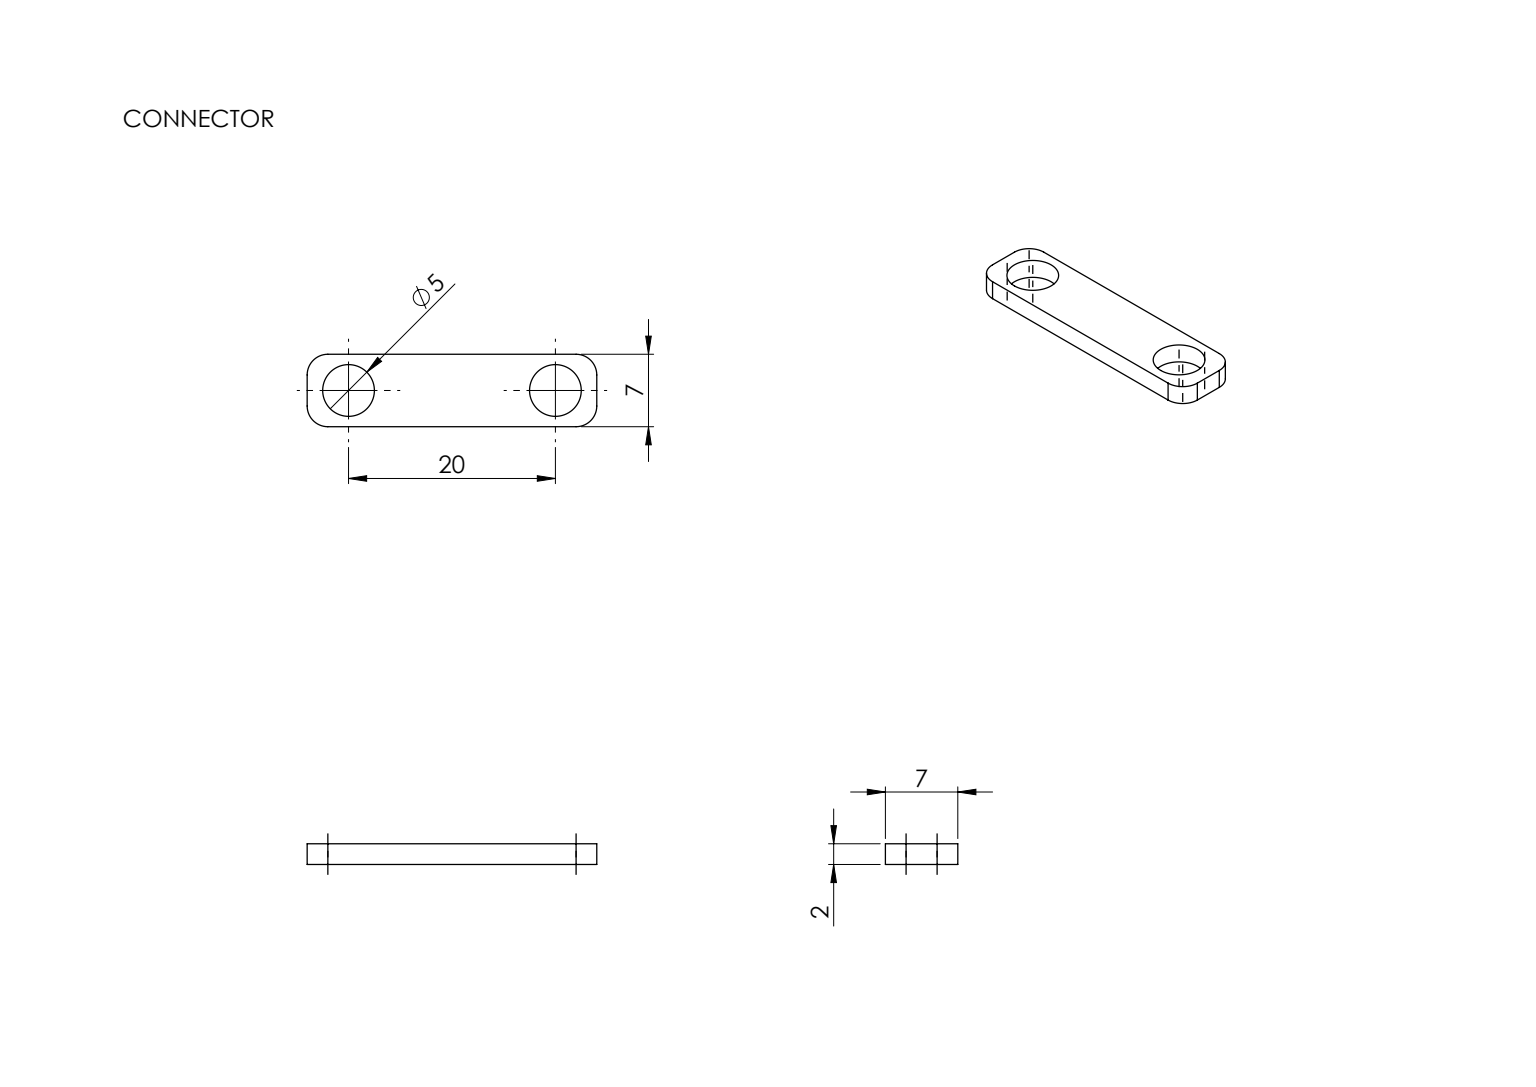
ISO-10303-21;
HEADER;
FILE_DESCRIPTION (('STEP AP214'),
    '1' );
FILE_NAME ('connector.step',
    '2026-10-08T13:56:24',
    ( '' ),
    ( '' ),
    'SwSTEP 2.0',
    'SolidWorks 2026',
    '' );
FILE_SCHEMA (( 'AUTOMOTIVE_DESIGN' ));
ENDSEC;

DATA;
#18=ADVANCED_FACE ( 'NONE', ( #40 ), #4954, .F. ) ;
#25=DIRECTION ( 'NONE',  ( -0.000000000000000000, -1.000000000000000000, -0.000000000000000000 ) ) ;
#35=LINE ( 'NONE', #1227, #14934 ) ;
#40=FACE_OUTER_BOUND ( 'NONE', #10361, .T. ) ;
#55=ORIENTED_EDGE ( 'NONE', *, *, #1011, .T. ) ;
#119=EDGE_CURVE ( 'NONE', #13173, #1506, #10244, .T. ) ;
#142=AXIS2_PLACEMENT_3D ( 'NONE', #6437, #6586, #9027 ) ;
#156=DIRECTION ( 'NONE',  ( 0.000000000000000000, 1.000000000000000000, -0.000000000000000000 ) ) ;
#158=ORIENTED_EDGE ( 'NONE', *, *, #11026, .F. ) ;
#174=PLANE ( 'NONE',  #5147 ) ;
#229=ORIENTED_EDGE ( 'NONE', *, *, #1759, .F. ) ;
#241=VECTOR ( 'NONE', #6289, 1000.000000000000000 ) ;
#307=VERTEX_POINT ( 'NONE', #7662 ) ;
#454=ORIENTED_EDGE ( 'NONE', *, *, #5990, .F. ) ;
#498=DIRECTION ( 'NONE',  ( 1.000000000000000000, 0.000000000000000000, 0.000000000000000000 ) ) ;
#522=VECTOR ( 'NONE', #25, 1000.000000000000000 ) ;
#523=FACE_OUTER_BOUND ( 'NONE', #7763, .T. ) ;
#595=FILL_AREA_STYLE_COLOUR ( '', #11712 ) ;
#608=ADVANCED_BREP_SHAPE_REPRESENTATION ( '', ( #9113, #3223 ), #1938 ) ;
#618=CARTESIAN_POINT ( 'NONE',  ( -17.99999999999979394, -11.00000000000000178, 1.499999999999999112 ) ) ;
#684=CIRCLE ( 'NONE', #4805, 2.000000000000000888 ) ;
#698=DIRECTION ( 'NONE',  ( 0.000000000000000000, 0.000000000000000000, 1.000000000000000000 ) ) ;
#724=AXIS2_PLACEMENT_3D ( 'NONE', #13932, #9982, #2858 ) ;
#756=PRESENTATION_STYLE_ASSIGNMENT (( #11957 ) ) ;
#763=ADVANCED_FACE ( 'NONE', ( #6395 ), #15112, .T. ) ;
#800=EDGE_CURVE ( 'NONE', #4542, #3229, #6635, .T. ) ;
#828=( NAMED_UNIT ( * ) PLANE_ANGLE_UNIT ( ) SI_UNIT ( $, .RADIAN. ) );
#835=CARTESIAN_POINT ( 'NONE',  ( -39.99999999999999289, -11.00000000000000178, 2.500000000001739497 ) ) ;
#849=ORIENTED_EDGE ( 'NONE', *, *, #13885, .T. ) ;
#862=FILL_AREA_STYLE_COLOUR ( '', #3052 ) ;
#897=ORIENTED_EDGE ( 'NONE', *, *, #7225, .T. ) ;
#914=CYLINDRICAL_SURFACE ( 'NONE', #5036, 2.500000000000909495 ) ;
#968=EDGE_LOOP ( 'NONE', ( #5323, #8194, #3762, #2718 ) ) ;
#1005=CYLINDRICAL_SURFACE ( 'NONE', #2041, 2.499999999999998668 ) ;
#1010=CARTESIAN_POINT ( 'NONE',  ( -19.99999999999956657, -11.00000000000000178, 8.786575603324269439E-13 ) ) ;
#1011=EDGE_CURVE ( 'NONE', #9125, #9091, #1099, .T. ) ;
#1051=LINE ( 'NONE', #12031, #10121 ) ;
#1087=SURFACE_SIDE_STYLE ('',( #12150 ) ) ;
#1099=CIRCLE ( 'NONE', #8348, 2.000000000000000888 ) ;
#1133=ORIENTED_EDGE ( 'NONE', *, *, #3684, .T. ) ;
#1158=CARTESIAN_POINT ( 'NONE',  ( -19.99999999999956657, -11.00000000000000178, -2.499999999999120259 ) ) ;
#1164=CARTESIAN_POINT ( 'NONE',  ( -15.99999999999979217, -9.000000000000001776, -1.500000000000001110 ) ) ;
#1180=EDGE_CURVE ( 'NONE', #9048, #13189, #4457, .T. ) ;
#1193=ORIENTED_EDGE ( 'NONE', *, *, #1975, .T. ) ;
#1227=CARTESIAN_POINT ( 'NONE',  ( -41.99999999999978684, -11.00000000000000178, 3.499999999999998668 ) ) ;
#1254=ORIENTED_EDGE ( 'NONE', *, *, #1180, .T. ) ;
#1305=DIRECTION ( 'NONE',  ( 0.000000000000000000, 0.000000000000000000, 1.000000000000000000 ) ) ;
#1385=CARTESIAN_POINT ( 'NONE',  ( -39.99999999999999289, -9.000000000000001776, 8.300651832549021947E-13 ) ) ;
#1476=VERTEX_POINT ( 'NONE', #4588 ) ;
#1506=VERTEX_POINT ( 'NONE', #15355 ) ;
#1518=VECTOR ( 'NONE', #3284, 1000.000000000000000 ) ;
#1677=CARTESIAN_POINT ( 'NONE',  ( -41.99999999999978684, -11.00000000000000178, 1.499999999999999112 ) ) ;
#1692=FACE_OUTER_BOUND ( 'NONE', #5404, .T. ) ;
#1707=DIRECTION ( 'NONE',  ( 0.000000000000000000, 0.000000000000000000, 1.000000000000000000 ) ) ;
#1759=EDGE_CURVE ( 'NONE', #1476, #14724, #14936, .T. ) ;
#1818=DIRECTION ( 'NONE',  ( 0.000000000000000000, 0.000000000000000000, -1.000000000000000000 ) ) ;
#1868=( NAMED_UNIT ( * ) SI_UNIT ( $, .STERADIAN. ) SOLID_ANGLE_UNIT ( ) );
#1880=CARTESIAN_POINT ( 'NONE',  ( -39.99999999999999289, -9.000000000000001776, -2.500000000000079492 ) ) ;
#1938=( GEOMETRIC_REPRESENTATION_CONTEXT ( 3 ) GLOBAL_UNCERTAINTY_ASSIGNED_CONTEXT ( ( #7400 ) ) GLOBAL_UNIT_ASSIGNED_CONTEXT ( ( #14406, #828, #1868 ) ) REPRESENTATION_CONTEXT ( 'NONE', 'WORKASPACE' ) );
#1957=APPLICATION_CONTEXT ( 'automotive_design' ) ;
#1961=VECTOR ( 'NONE', #15902, 1000.000000000000000 ) ;
#1974=ORIENTED_EDGE ( 'NONE', *, *, #5141, .T. ) ;
#1975=EDGE_CURVE ( 'NONE', #6779, #6035, #6277, .T. ) ;
#1985=CARTESIAN_POINT ( 'NONE',  ( -41.99999999999978684, -9.000000000000001776, 3.499999999999998668 ) ) ;
#2039=DIRECTION ( 'NONE',  ( 0.000000000000000000, 0.000000000000000000, 1.000000000000000000 ) ) ;
#2041=AXIS2_PLACEMENT_3D ( 'NONE', #9494, #3190, #14264 ) ;
#2057=ORIENTED_EDGE ( 'NONE', *, *, #7517, .T. ) ;
#2073=ORIENTED_EDGE ( 'NONE', *, *, #7225, .F. ) ;
#2109=ORIENTED_EDGE ( 'NONE', *, *, #5990, .T. ) ;
#2140=CARTESIAN_POINT ( 'NONE',  ( -17.99999999999979394, -9.000000000000001776, -3.500000000000000888 ) ) ;
#2146=EDGE_LOOP ( 'NONE', ( #849, #3533 ) ) ;
#2166=EDGE_LOOP ( 'NONE', ( #10473, #8805 ) ) ;
#2254=DIRECTION ( 'NONE',  ( 0.000000000000000000, 0.000000000000000000, 1.000000000000000000 ) ) ;
#2269=MECHANICAL_DESIGN_GEOMETRIC_PRESENTATION_REPRESENTATION('',(#9256),#10548);
#2317=LINE ( 'NONE', #3611, #13079 ) ;
#2336=CARTESIAN_POINT ( 'NONE',  ( -39.99999999999999289, -11.00000000000000178, 8.300651832549021947E-13 ) ) ;
#2350=EDGE_CURVE ( 'NONE', #307, #2847, #1051, .T. ) ;
#2464=CARTESIAN_POINT ( 'NONE',  ( -15.99999999999979217, -9.000000000000001776, -1.500000000000001110 ) ) ;
#2554=CARTESIAN_POINT ( 'NONE',  ( -41.99999999999978684, -11.00000000000000178, -3.500000000000001776 ) ) ;
#2659=EDGE_CURVE ( 'NONE', #2847, #3269, #15607, .T. ) ;
#2701=FACE_BOUND ( 'NONE', #2146, .T. ) ;
#2718=ORIENTED_EDGE ( 'NONE', *, *, #5141, .F. ) ;
#2728=CARTESIAN_POINT ( 'NONE',  ( -17.99999999999979394, -9.000000000000001776, 1.499999999999999112 ) ) ;
#2847=VERTEX_POINT ( 'NONE', #2554 ) ;
#2858=DIRECTION ( 'NONE',  ( 0.000000000000000000, 0.000000000000000000, 1.000000000000000000 ) ) ;
#2860=DIRECTION ( 'NONE',  ( 0.000000000000000000, -0.000000000000000000, 1.000000000000000000 ) ) ;
#2875=CARTESIAN_POINT ( 'NONE',  ( -15.99999999999979217, -11.00000000000000178, -1.500000000000001110 ) ) ;
#2886=ORIENTED_EDGE ( 'NONE', *, *, #14291, .F. ) ;
#2928=LINE ( 'NONE', #1880, #7434 ) ;
#2937=DIRECTION ( 'NONE',  ( 0.000000000000000000, 1.000000000000000000, 0.000000000000000000 ) ) ;
#2945=FACE_OUTER_BOUND ( 'NONE', #968, .T. ) ;
#3005=ORIENTED_EDGE ( 'NONE', *, *, #1011, .F. ) ;
#3013=CARTESIAN_POINT ( 'NONE',  ( -15.99999999999979217, -9.000000000000001776, -1.500000000000001110 ) ) ;
#3034=FACE_OUTER_BOUND ( 'NONE', #10178, .T. ) ;
#3052=COLOUR_RGB ( '', 0.40784314, 0.44705882, 0.49803922) ;
#3102=EDGE_CURVE ( 'NONE', #12397, #3134, #14026, .T. ) ;
#3110=DIRECTION ( 'NONE',  ( 1.000000000000000000, 0.000000000000000000, 0.000000000000000000 ) ) ;
#3134=VERTEX_POINT ( 'NONE', #10577 ) ;
#3190=DIRECTION ( 'NONE',  ( -0.000000000000000000, -1.000000000000000000, -0.000000000000000000 ) ) ;
#3223=AXIS2_PLACEMENT_3D ( 'NONE', #11897, #11972, #4638 ) ;
#3229=VERTEX_POINT ( 'NONE', #10485 ) ;
#3239=DIRECTION ( 'NONE',  ( 0.000000000000000000, 1.000000000000000000, -0.000000000000000000 ) ) ;
#3256=CYLINDRICAL_SURFACE ( 'NONE', #6862, 2.000000000000000888 ) ;
#3269=VERTEX_POINT ( 'NONE', #12966 ) ;
#3276=CARTESIAN_POINT ( 'NONE',  ( -39.99999999999999289, -9.000000000000001776, 8.300651832549021947E-13 ) ) ;
#3284=DIRECTION ( 'NONE',  ( -0.000000000000000000, -1.000000000000000000, -0.000000000000000000 ) ) ;
#3332=ADVANCED_FACE ( 'NONE', ( #7249 ), #12072, .F. ) ;
#3402=FILL_AREA_STYLE ('',( #595 ) ) ;
#3413=DIRECTION ( 'NONE',  ( -0.000000000000000000, -1.000000000000000000, -0.000000000000000000 ) ) ;
#3428=DIRECTION ( 'NONE',  ( 0.000000000000000000, 1.000000000000000000, 0.000000000000000000 ) ) ;
#3469=DIRECTION ( 'NONE',  ( -1.000000000000000000, -0.000000000000000000, -0.000000000000000000 ) ) ;
#3499=DIRECTION ( 'NONE',  ( 0.000000000000000000, 0.000000000000000000, 1.000000000000000000 ) ) ;
#3518=AXIS2_PLACEMENT_3D ( 'NONE', #7554, #14986, #4060 ) ;
#3533=ORIENTED_EDGE ( 'NONE', *, *, #5671, .T. ) ;
#3607=LINE ( 'NONE', #7100, #1961 ) ;
#3611=CARTESIAN_POINT ( 'NONE',  ( -15.99999999999979217, -9.000000000000001776, -1.500000000000001110 ) ) ;
#3684=EDGE_CURVE ( 'NONE', #10705, #12397, #9407, .T. ) ;
#3762=ORIENTED_EDGE ( 'NONE', *, *, #14528, .F. ) ;
#3786=VECTOR ( 'NONE', #7903, 1000.000000000000000 ) ;
#3809=CIRCLE ( 'NONE', #724, 2.000000000000000888 ) ;
#3810=ADVANCED_FACE ( 'NONE', ( #7468, #13914, #7548 ), #3892, .T. ) ;
#3833=PRODUCT_DEFINITION_CONTEXT ( 'detailed design', #1957, 'design' ) ;
#3846=ORIENTED_EDGE ( 'NONE', *, *, #7499, .T. ) ;
#3872=CYLINDRICAL_SURFACE ( 'NONE', #14600, 2.000000000000000888 ) ;
#3892=PLANE ( 'NONE',  #8955 ) ;
#3893=DIRECTION ( 'NONE',  ( -0.000000000000000000, -1.000000000000000000, -0.000000000000000000 ) ) ;
#3897=CARTESIAN_POINT ( 'NONE',  ( -41.99999999999978684, -9.000000000000001776, 3.499999999999998668 ) ) ;
#3902=EDGE_CURVE ( 'NONE', #6035, #6779, #12054, .T. ) ;
#3941=DIRECTION ( 'NONE',  ( 0.000000000000000000, 0.000000000000000000, 1.000000000000000000 ) ) ;
#4031=ADVANCED_FACE ( 'NONE', ( #523 ), #5678, .T. ) ;
#4046=LINE ( 'NONE', #8917, #4614 ) ;
#4060=DIRECTION ( 'NONE',  ( 0.000000000000000000, 0.000000000000000000, 1.000000000000000000 ) ) ;
#4065=FACE_OUTER_BOUND ( 'NONE', #7295, .T. ) ;
#4156=FACE_BOUND ( 'NONE', #2166, .T. ) ;
#4179=UNCERTAINTY_MEASURE_WITH_UNIT (LENGTH_MEASURE( 1.000000000000000082E-05 ), #14586, 'distance_accuracy_value', 'NONE');
#4242=ORIENTED_EDGE ( 'NONE', *, *, #13940, .F. ) ;
#4263=AXIS2_PLACEMENT_3D ( 'NONE', #618, #2937, #2860 ) ;
#4292=ORIENTED_EDGE ( 'NONE', *, *, #3102, .T. ) ;
#4381=EDGE_CURVE ( 'NONE', #9125, #14724, #2317, .T. ) ;
#4410=ORIENTED_EDGE ( 'NONE', *, *, #9663, .F. ) ;
#4419=CARTESIAN_POINT ( 'NONE',  ( -19.99999999999956657, -9.000000000000001776, -2.499999999999120259 ) ) ;
#4426=ORIENTED_EDGE ( 'NONE', *, *, #800, .T. ) ;
#4457=CIRCLE ( 'NONE', #11675, 2.499999999999998668 ) ;
#4466=ORIENTED_EDGE ( 'NONE', *, *, #7538, .F. ) ;
#4528=AXIS2_PLACEMENT_3D ( 'NONE', #15021, #156, #9842 ) ;
#4542=VERTEX_POINT ( 'NONE', #12721 ) ;
#4588=CARTESIAN_POINT ( 'NONE',  ( -15.99999999999979217, -11.00000000000000178, 1.499999999999998890 ) ) ;
#4602=EDGE_CURVE ( 'NONE', #9091, #13173, #9194, .T. ) ;
#4614=VECTOR ( 'NONE', #1707, 1000.000000000000000 ) ;
#4619=AXIS2_PLACEMENT_3D ( 'NONE', #5093, #12506, #6633 ) ;
#4622=SURFACE_SIDE_STYLE ('',( #5519 ) ) ;
#4638=DIRECTION ( 'NONE',  ( 1.000000000000000000, 0.000000000000000000, 0.000000000000000000 ) ) ;
#4656=ORIENTED_EDGE ( 'NONE', *, *, #7809, .T. ) ;
#4735=ORIENTED_EDGE ( 'NONE', *, *, #9375, .F. ) ;
#4783=CIRCLE ( 'NONE', #5813, 2.499999999999998668 ) ;
#4784=CARTESIAN_POINT ( 'NONE',  ( -39.99999999999999289, -9.000000000000001776, 8.300651832549021947E-13 ) ) ;
#4805=AXIS2_PLACEMENT_3D ( 'NONE', #1677, #8808, #3941 ) ;
#4866=CIRCLE ( 'NONE', #15198, 2.500000000000909495 ) ;
#4878=DIRECTION ( 'NONE',  ( 1.000000000000000000, 0.000000000000000000, 0.000000000000000000 ) ) ;
#4954=CYLINDRICAL_SURFACE ( 'NONE', #8447, 2.499999999999998668 ) ;
#4984=CARTESIAN_POINT ( 'NONE',  ( -17.99999999999979394, -9.000000000000001776, -3.500000000000000888 ) ) ;
#5036=AXIS2_PLACEMENT_3D ( 'NONE', #4784, #5756, #7297 ) ;
#5093=CARTESIAN_POINT ( 'NONE',  ( -17.99999999999979394, -11.00000000000000178, 1.499999999999999112 ) ) ;
#5141=EDGE_CURVE ( 'NONE', #6035, #9656, #2928, .T. ) ;
#5147=AXIS2_PLACEMENT_3D ( 'NONE', #5421, #498, #10274 ) ;
#5156=LINE ( 'NONE', #11441, #241 ) ;
#5227=AXIS2_PLACEMENT_3D ( 'NONE', #6476, #7697, #10426 ) ;
#5253=DIRECTION ( 'NONE',  ( -0.000000000000000000, -1.000000000000000000, -0.000000000000000000 ) ) ;
#5297=ORIENTED_EDGE ( 'NONE', *, *, #1180, .F. ) ;
#5323=ORIENTED_EDGE ( 'NONE', *, *, #3902, .T. ) ;
#5404=EDGE_LOOP ( 'NONE', ( #897, #6728, #8945, #4656 ) ) ;
#5421=CARTESIAN_POINT ( 'NONE',  ( -43.99999999999978684, -9.000000000000001776, -1.500000000000000666 ) ) ;
#5429=ORIENTED_EDGE ( 'NONE', *, *, #7499, .F. ) ;
#5431=VERTEX_POINT ( 'NONE', #8148 ) ;
#5433=EDGE_CURVE ( 'NONE', #10705, #11234, #13045, .T. ) ;
#5440=DIRECTION ( 'NONE',  ( -0.000000000000000000, -1.000000000000000000, -0.000000000000000000 ) ) ;
#5481=ORIENTED_EDGE ( 'NONE', *, *, #9501, .T. ) ;
#5516=CARTESIAN_POINT ( 'NONE',  ( -41.99999999999978684, -9.000000000000001776, -1.500000000000000888 ) ) ;
#5519=SURFACE_STYLE_FILL_AREA ( #3402 ) ;
#5542=ORIENTED_EDGE ( 'NONE', *, *, #13940, .T. ) ;
#5617=CARTESIAN_POINT ( 'NONE',  ( -39.99999999999999289, -9.000000000000001776, -2.500000000000079492 ) ) ;
#5624=DIRECTION ( 'NONE',  ( 1.000000000000000000, 0.000000000000000000, -0.000000000000000000 ) ) ;
#5671=EDGE_CURVE ( 'NONE', #11827, #6744, #9496, .T. ) ;
#5678=CYLINDRICAL_SURFACE ( 'NONE', #14145, 2.000000000000000888 ) ;
#5756=DIRECTION ( 'NONE',  ( -0.000000000000000000, -1.000000000000000000, -0.000000000000000000 ) ) ;
#5813=AXIS2_PLACEMENT_3D ( 'NONE', #8537, #14577, #3499 ) ;
#5832=SHAPE_REPRESENTATION_RELATIONSHIP ( 'NONE' , 'NONE' ,  #15130, #608 ) ;
#5843=AXIS2_PLACEMENT_3D ( 'NONE', #3276, #6764, #1818 ) ;
#5906=VECTOR ( 'NONE', #3893, 1000.000000000000000 ) ;
#5910=AXIS2_PLACEMENT_3D ( 'NONE', #14748, #13275, #8618 ) ;
#5990=EDGE_CURVE ( 'NONE', #4542, #10705, #3809, .T. ) ;
#6027=( NAMED_UNIT ( * ) SI_UNIT ( $, .STERADIAN. ) SOLID_ANGLE_UNIT ( ) );
#6035=VERTEX_POINT ( 'NONE', #5617 ) ;
#6036=PRODUCT ( 'connector', 'connector', '', ( #7465 ) ) ;
#6108=PRESENTATION_STYLE_ASSIGNMENT (( #10870 ) ) ;
#6186=DIRECTION ( 'NONE',  ( 0.000000000000000000, 0.000000000000000000, 1.000000000000000000 ) ) ;
#6237=EDGE_CURVE ( 'NONE', #11234, #3134, #35, .T. ) ;
#6251=DIRECTION ( 'NONE',  ( 0.000000000000000000, -0.000000000000000000, 1.000000000000000000 ) ) ;
#6276=EDGE_LOOP ( 'NONE', ( #15549, #12998, #5429, #5481 ) ) ;
#6277=CIRCLE ( 'NONE', #15310, 2.500000000000909495 ) ;
#6289=DIRECTION ( 'NONE',  ( -0.000000000000000000, -1.000000000000000000, -0.000000000000000000 ) ) ;
#6395=FACE_OUTER_BOUND ( 'NONE', #14036, .T. ) ;
#6408=AXIS2_PLACEMENT_3D ( 'NONE', #1385, #13740, #1305 ) ;
#6437=CARTESIAN_POINT ( 'NONE',  ( -39.99999999999999289, -11.00000000000000178, 8.300651832549021947E-13 ) ) ;
#6476=CARTESIAN_POINT ( 'NONE',  ( -41.99999999999978684, -9.000000000000001776, 1.499999999999999112 ) ) ;
#6516=EDGE_LOOP ( 'NONE', ( #5297, #4242 ) ) ;
#6529=VECTOR ( 'NONE', #14023, 1000.000000000000000 ) ;
#6586=DIRECTION ( 'NONE',  ( 0.000000000000000000, 1.000000000000000000, 0.000000000000000000 ) ) ;
#6607=DIRECTION ( 'NONE',  ( -0.000000000000000000, -1.000000000000000000, -0.000000000000000000 ) ) ;
#6624=DIRECTION ( 'NONE',  ( -0.000000000000000000, -1.000000000000000000, -0.000000000000000000 ) ) ;
#6633=DIRECTION ( 'NONE',  ( 0.000000000000000000, 0.000000000000000000, 1.000000000000000000 ) ) ;
#6635=LINE ( 'NONE', #13896, #12964 ) ;
#6668=PLANE ( 'NONE',  #12255 ) ;
#6723=PRODUCT_DEFINITION ( 'UNKNOWN', '', #8973, #3833 ) ;
#6728=ORIENTED_EDGE ( 'NONE', *, *, #800, .F. ) ;
#6744=VERTEX_POINT ( 'NONE', #1158 ) ;
#6764=DIRECTION ( 'NONE',  ( -0.000000000000000000, -1.000000000000000000, -0.000000000000000000 ) ) ;
#6779=VERTEX_POINT ( 'NONE', #11029 ) ;
#6811=ORIENTED_EDGE ( 'NONE', *, *, #4602, .F. ) ;
#6812=( NAMED_UNIT ( * ) PLANE_ANGLE_UNIT ( ) SI_UNIT ( $, .RADIAN. ) );
#6831=ORIENTED_EDGE ( 'NONE', *, *, #9501, .F. ) ;
#6833=ORIENTED_EDGE ( 'NONE', *, *, #2350, .T. ) ;
#6862=AXIS2_PLACEMENT_3D ( 'NONE', #11494, #15552, #10620 ) ;
#6904=DIRECTION ( 'NONE',  ( 0.000000000000000000, 0.000000000000000000, 1.000000000000000000 ) ) ;
#6931=DIRECTION ( 'NONE',  ( -0.000000000000000000, -1.000000000000000000, -0.000000000000000000 ) ) ;
#6945=ORIENTED_EDGE ( 'NONE', *, *, #5671, .F. ) ;
#6965=VERTEX_POINT ( 'NONE', #835 ) ;
#6995=ORIENTED_EDGE ( 'NONE', *, *, #11649, .T. ) ;
#6998=EDGE_LOOP ( 'NONE', ( #1254, #7541, #7678, #4735 ) ) ;
#7009=CARTESIAN_POINT ( 'NONE',  ( -43.99999999999978684, -9.000000000000001776, -1.500000000000000666 ) ) ;
#7095=ORIENTED_EDGE ( 'NONE', *, *, #5433, .T. ) ;
#7100=CARTESIAN_POINT ( 'NONE',  ( -39.99999999999999289, -9.000000000000001776, 2.500000000001739497 ) ) ;
#7199=ORIENTED_EDGE ( 'NONE', *, *, #119, .F. ) ;
#7225=EDGE_CURVE ( 'NONE', #3269, #3229, #4046, .T. ) ;
#7240=DIRECTION ( 'NONE',  ( 0.000000000000000000, 0.000000000000000000, -1.000000000000000000 ) ) ;
#7249=FACE_OUTER_BOUND ( 'NONE', #12934, .T. ) ;
#7295=EDGE_LOOP ( 'NONE', ( #10431, #4466, #3005, #10115 ) ) ;
#7297=DIRECTION ( 'NONE',  ( 0.000000000000000000, 0.000000000000000000, -1.000000000000000000 ) ) ;
#7308=ORIENTED_EDGE ( 'NONE', *, *, #3902, .F. ) ;
#7400=UNCERTAINTY_MEASURE_WITH_UNIT (LENGTH_MEASURE( 1.000000000000000082E-05 ), #14406, 'distance_accuracy_value', 'NONE');
#7412=AXIS2_PLACEMENT_3D ( 'NONE', #12884, #698, #5624 ) ;
#7434=VECTOR ( 'NONE', #12943, 1000.000000000000000 ) ;
#7465=PRODUCT_CONTEXT ( 'NONE', #15891, 'mechanical' ) ;
#7468=FACE_BOUND ( 'NONE', #6516, .T. ) ;
#7499=EDGE_CURVE ( 'NONE', #5431, #9125, #7756, .T. ) ;
#7505=DIRECTION ( 'NONE',  ( -0.000000000000000000, -1.000000000000000000, -0.000000000000000000 ) ) ;
#7517=EDGE_CURVE ( 'NONE', #13173, #2847, #5156, .T. ) ;
#7538=EDGE_CURVE ( 'NONE', #9091, #307, #11125, .T. ) ;
#7541=ORIENTED_EDGE ( 'NONE', *, *, #11026, .T. ) ;
#7548=FACE_BOUND ( 'NONE', #14813, .T. ) ;
#7554=CARTESIAN_POINT ( 'NONE',  ( -41.99999999999978684, -9.000000000000001776, -1.500000000000000888 ) ) ;
#7662=CARTESIAN_POINT ( 'NONE',  ( -17.99999999999979394, -11.00000000000000178, -3.500000000000000888 ) ) ;
#7678=ORIENTED_EDGE ( 'NONE', *, *, #13885, .F. ) ;
#7697=DIRECTION ( 'NONE',  ( -0.000000000000000000, -1.000000000000000000, -0.000000000000000000 ) ) ;
#7756=LINE ( 'NONE', #2464, #10309 ) ;
#7763=EDGE_LOOP ( 'NONE', ( #11409, #14077, #7199, #2057 ) ) ;
#7785=ORIENTED_EDGE ( 'NONE', *, *, #1975, .F. ) ;
#7809=EDGE_CURVE ( 'NONE', #1506, #3269, #14507, .T. ) ;
#7843=FACE_OUTER_BOUND ( 'NONE', #11219, .T. ) ;
#7889=CIRCLE ( 'NONE', #14071, 2.000000000000000888 ) ;
#7903=DIRECTION ( 'NONE',  ( -1.000000000000000000, -0.000000000000000000, -0.000000000000000000 ) ) ;
#7981=PLANE ( 'NONE',  #7412 ) ;
#7992=CIRCLE ( 'NONE', #4619, 2.000000000000000888 ) ;
#8148=CARTESIAN_POINT ( 'NONE',  ( -15.99999999999979217, -9.000000000000001776, 1.499999999999998890 ) ) ;
#8187=CARTESIAN_POINT ( 'NONE',  ( -17.99999999999979394, -9.000000000000001776, -1.500000000000000888 ) ) ;
#8194=ORIENTED_EDGE ( 'NONE', *, *, #12013, .T. ) ;
#8259=CARTESIAN_POINT ( 'NONE',  ( -41.99999999999978684, -11.00000000000000178, -1.500000000000000888 ) ) ;
#8262=ORIENTED_EDGE ( 'NONE', *, *, #6237, .F. ) ;
#8327=EDGE_CURVE ( 'NONE', #3134, #1476, #7992, .T. ) ;
#8348=AXIS2_PLACEMENT_3D ( 'NONE', #8187, #3239, #11793 ) ;
#8354=ADVANCED_FACE ( 'NONE', ( #1692 ), #174, .F. ) ;
#8399=CIRCLE ( 'NONE', #14572, 2.499999999999998668 ) ;
#8440=DIRECTION ( 'NONE',  ( 0.000000000000000000, 1.000000000000000000, 0.000000000000000000 ) ) ;
#8447=AXIS2_PLACEMENT_3D ( 'NONE', #8454, #13349, #7240 ) ;
#8454=CARTESIAN_POINT ( 'NONE',  ( -19.99999999999956657, -9.000000000000001776, 8.786575603324269439E-13 ) ) ;
#8537=CARTESIAN_POINT ( 'NONE',  ( -19.99999999999956657, -9.000000000000001776, 8.786575603324269439E-13 ) ) ;
#8588=ORIENTED_EDGE ( 'NONE', *, *, #14291, .T. ) ;
#8618=DIRECTION ( 'NONE',  ( -1.000000000000000000, 0.000000000000000000, -0.000000000000000000 ) ) ;
#8632=STYLED_ITEM ( 'NONE', ( #756 ), #608 ) ;
#8667=ORIENTED_EDGE ( 'NONE', *, *, #7538, .T. ) ;
#8783=ORIENTED_EDGE ( 'NONE', *, *, #4602, .T. ) ;
#8805=ORIENTED_EDGE ( 'NONE', *, *, #9663, .T. ) ;
#8808=DIRECTION ( 'NONE',  ( 0.000000000000000000, 1.000000000000000000, 0.000000000000000000 ) ) ;
#8810=DIRECTION ( 'NONE',  ( 0.000000000000000000, 0.000000000000000000, -1.000000000000000000 ) ) ;
#8890=MECHANICAL_DESIGN_GEOMETRIC_PRESENTATION_REPRESENTATION('',(#8632),#12213);
#8917=CARTESIAN_POINT ( 'NONE',  ( -43.99999999999978684, -11.00000000000000178, -1.500000000000000666 ) ) ;
#8931=CIRCLE ( 'NONE', #4528, 2.000000000000000888 ) ;
#8945=ORIENTED_EDGE ( 'NONE', *, *, #15905, .F. ) ;
#8955=AXIS2_PLACEMENT_3D ( 'NONE', #12687, #13578, #6251 ) ;
#8973=PRODUCT_DEFINITION_FORMATION_WITH_SPECIFIED_SOURCE ( 'ANY', '', #6036, .NOT_KNOWN. ) ;
#9023=UNCERTAINTY_MEASURE_WITH_UNIT (LENGTH_MEASURE( 1.000000000000000082E-05 ), #15383, 'distance_accuracy_value', 'NONE');
#9027=DIRECTION ( 'NONE',  ( 0.000000000000000000, 0.000000000000000000, 1.000000000000000000 ) ) ;
#9044=CARTESIAN_POINT ( 'NONE',  ( -17.99999999999979394, -9.000000000000001776, 3.499999999999998668 ) ) ;
#9048=VERTEX_POINT ( 'NONE', #4419 ) ;
#9091=VERTEX_POINT ( 'NONE', #2140 ) ;
#9113=MANIFOLD_SOLID_BREP ( 'Boss-Extrude1', #13832 ) ;
#9125=VERTEX_POINT ( 'NONE', #1164 ) ;
#9133=CARTESIAN_POINT ( 'NONE',  ( -41.99999999999978684, -9.000000000000001776, -3.500000000000001776 ) ) ;
#9194=LINE ( 'NONE', #14199, #3786 ) ;
#9256=STYLED_ITEM ( 'NONE', ( #6108 ), #9113 ) ;
#9268=ORIENTED_EDGE ( 'NONE', *, *, #6237, .T. ) ;
#9340=FACE_OUTER_BOUND ( 'NONE', #6998, .T. ) ;
#9375=EDGE_CURVE ( 'NONE', #9048, #6744, #10699, .T. ) ;
#9407=LINE ( 'NONE', #14183, #11399 ) ;
#9417=ORIENTED_EDGE ( 'NONE', *, *, #7517, .F. ) ;
#9448=DIRECTION ( 'NONE',  ( 0.000000000000000000, 1.000000000000000000, 0.000000000000000000 ) ) ;
#9473=( NAMED_UNIT ( * ) SI_UNIT ( $, .STERADIAN. ) SOLID_ANGLE_UNIT ( ) );
#9488=CARTESIAN_POINT ( 'NONE',  ( -19.99999999999956657, -9.000000000000001776, -2.499999999999120259 ) ) ;
#9494=CARTESIAN_POINT ( 'NONE',  ( -19.99999999999956657, -9.000000000000001776, 8.786575603324269439E-13 ) ) ;
#9496=CIRCLE ( 'NONE', #11799, 2.499999999999998668 ) ;
#9501=EDGE_CURVE ( 'NONE', #5431, #1476, #9877, .T. ) ;
#9574=DIRECTION ( 'NONE',  ( 0.000000000000000000, 0.000000000000000000, 1.000000000000000000 ) ) ;
#9624=VECTOR ( 'NONE', #6607, 1000.000000000000000 ) ;
#9656=VERTEX_POINT ( 'NONE', #10987 ) ;
#9663=EDGE_CURVE ( 'NONE', #6965, #9656, #4866, .T. ) ;
#9675=ORIENTED_EDGE ( 'NONE', *, *, #12013, .F. ) ;
#9732=CARTESIAN_POINT ( 'NONE',  ( -39.99999999999999289, -9.000000000000001776, 8.300651832549021947E-13 ) ) ;
#9842=DIRECTION ( 'NONE',  ( 0.000000000000000000, 0.000000000000000000, -1.000000000000000000 ) ) ;
#9865=LINE ( 'NONE', #11088, #522 ) ;
#9877=LINE ( 'NONE', #13579, #5906 ) ;
#9933=CIRCLE ( 'NONE', #142, 2.500000000000909495 ) ;
#9966=ORIENTED_EDGE ( 'NONE', *, *, #2659, .F. ) ;
#9982=DIRECTION ( 'NONE',  ( 0.000000000000000000, 1.000000000000000000, 0.000000000000000000 ) ) ;
#10037=CARTESIAN_POINT ( 'NONE',  ( -41.99999999999978684, -11.00000000000000178, 3.499999999999998668 ) ) ;
#10115=ORIENTED_EDGE ( 'NONE', *, *, #4381, .T. ) ;
#10121=VECTOR ( 'NONE', #3469, 1000.000000000000000 ) ;
#10178=EDGE_LOOP ( 'NONE', ( #6833, #9417, #6811, #8667 ) ) ;
#10214=ORIENTED_EDGE ( 'NONE', *, *, #9375, .T. ) ;
#10244=CIRCLE ( 'NONE', #3518, 2.000000000000000888 ) ;
#10274=DIRECTION ( 'NONE',  ( 0.000000000000000000, 0.000000000000000000, -1.000000000000000000 ) ) ;
#10308=FACE_OUTER_BOUND ( 'NONE', #6276, .T. ) ;
#10309=VECTOR ( 'NONE', #14849, 1000.000000000000000 ) ;
#10361=EDGE_LOOP ( 'NONE', ( #158, #5542, #10214, #6945 ) ) ;
#10426=DIRECTION ( 'NONE',  ( 0.000000000000000000, 0.000000000000000000, -1.000000000000000000 ) ) ;
#10431=ORIENTED_EDGE ( 'NONE', *, *, #15217, .T. ) ;
#10473=ORIENTED_EDGE ( 'NONE', *, *, #14528, .T. ) ;
#10485=CARTESIAN_POINT ( 'NONE',  ( -43.99999999999978684, -11.00000000000000178, 1.499999999999998668 ) ) ;
#10512=DIRECTION ( 'NONE',  ( 0.000000000000000000, 0.000000000000000000, 1.000000000000000000 ) ) ;
#10546=ADVANCED_FACE ( 'NONE', ( #9340 ), #1005, .F. ) ;
#10548=( GEOMETRIC_REPRESENTATION_CONTEXT ( 3 ) GLOBAL_UNCERTAINTY_ASSIGNED_CONTEXT ( ( #4179 ) ) GLOBAL_UNIT_ASSIGNED_CONTEXT ( ( #14586, #14673, #6027 ) ) REPRESENTATION_CONTEXT ( 'NONE', 'WORKASPACE' ) );
#10577=CARTESIAN_POINT ( 'NONE',  ( -17.99999999999979394, -11.00000000000000178, 3.499999999999998668 ) ) ;
#10620=DIRECTION ( 'NONE',  ( 0.000000000000000000, 0.000000000000000000, -1.000000000000000000 ) ) ;
#10684=DIRECTION ( 'NONE',  ( 0.000000000000000000, 0.000000000000000000, 1.000000000000000000 ) ) ;
#10699=LINE ( 'NONE', #9488, #13890 ) ;
#10705=VERTEX_POINT ( 'NONE', #3897 ) ;
#10764=DIRECTION ( 'NONE',  ( 0.000000000000000000, 1.000000000000000000, 0.000000000000000000 ) ) ;
#10804=ORIENTED_EDGE ( 'NONE', *, *, #8327, .F. ) ;
#10859=EDGE_LOOP ( 'NONE', ( #10804, #8262, #13158, #2073, #9966, #14230, #12597, #229 ) ) ;
#10870=SURFACE_STYLE_USAGE ( .BOTH. , #1087 ) ;
#10987=CARTESIAN_POINT ( 'NONE',  ( -39.99999999999999289, -11.00000000000000178, -2.500000000000079492 ) ) ;
#11026=EDGE_CURVE ( 'NONE', #13189, #11827, #9865, .T. ) ;
#11029=CARTESIAN_POINT ( 'NONE',  ( -39.99999999999999289, -9.000000000000001776, 2.500000000001739497 ) ) ;
#11031=VECTOR ( 'NONE', #6931, 1000.000000000000000 ) ;
#11077=DIRECTION ( 'NONE',  ( 0.000000000000000000, 1.000000000000000000, 0.000000000000000000 ) ) ;
#11088=CARTESIAN_POINT ( 'NONE',  ( -19.99999999999956657, -9.000000000000001776, 2.500000000000877520 ) ) ;
#11125=LINE ( 'NONE', #4984, #13122 ) ;
#11163=SHAPE_DEFINITION_REPRESENTATION ( #13373, #15130 ) ;
#11219=EDGE_LOOP ( 'NONE', ( #11502, #6831, #2886, #4292 ) ) ;
#11234=VERTEX_POINT ( 'NONE', #10037 ) ;
#11399=VECTOR ( 'NONE', #3110, 1000.000000000000000 ) ;
#11407=ORIENTED_EDGE ( 'NONE', *, *, #3684, .F. ) ;
#11409=ORIENTED_EDGE ( 'NONE', *, *, #2659, .T. ) ;
#11441=CARTESIAN_POINT ( 'NONE',  ( -41.99999999999978684, -9.000000000000001776, -3.500000000000001776 ) ) ;
#11494=CARTESIAN_POINT ( 'NONE',  ( -17.99999999999979394, -9.000000000000001776, -1.500000000000000888 ) ) ;
#11502=ORIENTED_EDGE ( 'NONE', *, *, #8327, .T. ) ;
#11649=EDGE_CURVE ( 'NONE', #3229, #11234, #684, .T. ) ;
#11675=AXIS2_PLACEMENT_3D ( 'NONE', #14546, #11077, #14630 ) ;
#11702=ORIENTED_EDGE ( 'NONE', *, *, #5433, .F. ) ;
#11712=COLOUR_RGB ( '', 0.40784314, 0.44705882, 0.49803922) ;
#11793=DIRECTION ( 'NONE',  ( 0.000000000000000000, 0.000000000000000000, -1.000000000000000000 ) ) ;
#11799=AXIS2_PLACEMENT_3D ( 'NONE', #12119, #10764, #10684 ) ;
#11827=VERTEX_POINT ( 'NONE', #15349 ) ;
#11897=CARTESIAN_POINT ( 'NONE',  ( 0.000000000000000000, 0.000000000000000000, 0.000000000000000000 ) ) ;
#11957=SURFACE_STYLE_USAGE ( .BOTH. , #4622 ) ;
#11963=AXIS2_PLACEMENT_3D ( 'NONE', #8259, #9448, #10512 ) ;
#11972=DIRECTION ( 'NONE',  ( 0.000000000000000000, 0.000000000000000000, 1.000000000000000000 ) ) ;
#11975=EDGE_LOOP ( 'NONE', ( #8588, #3846, #55, #8783, #13742, #15527, #2109, #1133 ) ) ;
#12013=EDGE_CURVE ( 'NONE', #6779, #6965, #3607, .T. ) ;
#12031=CARTESIAN_POINT ( 'NONE',  ( -41.99999999999978684, -11.00000000000000178, -3.500000000000000888 ) ) ;
#12054=CIRCLE ( 'NONE', #6408, 2.500000000000909495 ) ;
#12072=PLANE ( 'NONE',  #5910 ) ;
#12119=CARTESIAN_POINT ( 'NONE',  ( -19.99999999999956657, -11.00000000000000178, 8.786575603324269439E-13 ) ) ;
#12150=SURFACE_STYLE_FILL_AREA ( #12286 ) ;
#12192=CARTESIAN_POINT ( 'NONE',  ( -15.99999999999979217, -11.00000000000000178, -1.500000000000001110 ) ) ;
#12213=( GEOMETRIC_REPRESENTATION_CONTEXT ( 3 ) GLOBAL_UNCERTAINTY_ASSIGNED_CONTEXT ( ( #9023 ) ) GLOBAL_UNIT_ASSIGNED_CONTEXT ( ( #15383, #6812, #9473 ) ) REPRESENTATION_CONTEXT ( 'NONE', 'WORKASPACE' ) );
#12255=AXIS2_PLACEMENT_3D ( 'NONE', #3013, #13997, #6904 ) ;
#12286=FILL_AREA_STYLE ('',( #862 ) ) ;
#12348=ADVANCED_FACE ( 'NONE', ( #3034 ), #7981, .F. ) ;
#12367=ADVANCED_FACE ( 'NONE', ( #2945 ), #14347, .F. ) ;
#12397=VERTEX_POINT ( 'NONE', #12796 ) ;
#12506=DIRECTION ( 'NONE',  ( 0.000000000000000000, 1.000000000000000000, 0.000000000000000000 ) ) ;
#12597=ORIENTED_EDGE ( 'NONE', *, *, #15217, .F. ) ;
#12687=CARTESIAN_POINT ( 'NONE',  ( -17.99999999999979394, -9.000000000000001776, 1.499999999999999112 ) ) ;
#12721=CARTESIAN_POINT ( 'NONE',  ( -43.99999999999978684, -9.000000000000001776, 1.499999999999998668 ) ) ;
#12759=VECTOR ( 'NONE', #15487, 1000.000000000000000 ) ;
#12796=CARTESIAN_POINT ( 'NONE',  ( -17.99999999999979394, -9.000000000000001776, 3.499999999999998668 ) ) ;
#12822=CARTESIAN_POINT ( 'NONE',  ( -19.99999999999956657, -9.000000000000001776, 2.500000000000877520 ) ) ;
#12884=CARTESIAN_POINT ( 'NONE',  ( -41.99999999999978684, -9.000000000000001776, -3.500000000000000888 ) ) ;
#12934=EDGE_LOOP ( 'NONE', ( #9268, #13629, #11407, #7095 ) ) ;
#12943=DIRECTION ( 'NONE',  ( -0.000000000000000000, -1.000000000000000000, -0.000000000000000000 ) ) ;
#12964=VECTOR ( 'NONE', #5253, 1000.000000000000000 ) ;
#12966=CARTESIAN_POINT ( 'NONE',  ( -43.99999999999978684, -11.00000000000000178, -1.500000000000000666 ) ) ;
#12998=ORIENTED_EDGE ( 'NONE', *, *, #4381, .F. ) ;
#13009=DIRECTION ( 'NONE',  ( 0.000000000000000000, 0.000000000000000000, -1.000000000000000000 ) ) ;
#13045=LINE ( 'NONE', #1985, #11031 ) ;
#13079=VECTOR ( 'NONE', #13527, 1000.000000000000000 ) ;
#13122=VECTOR ( 'NONE', #7505, 1000.000000000000000 ) ;
#13134=ADVANCED_FACE ( 'NONE', ( #7843 ), #3872, .T. ) ;
#13158=ORIENTED_EDGE ( 'NONE', *, *, #11649, .F. ) ;
#13173=VERTEX_POINT ( 'NONE', #9133 ) ;
#13189=VERTEX_POINT ( 'NONE', #12822 ) ;
#13250=CARTESIAN_POINT ( 'NONE',  ( -17.99999999999979394, -9.000000000000001776, 1.499999999999999112 ) ) ;
#13275=DIRECTION ( 'NONE',  ( 0.000000000000000000, 0.000000000000000000, -1.000000000000000000 ) ) ;
#13349=DIRECTION ( 'NONE',  ( -0.000000000000000000, -1.000000000000000000, -0.000000000000000000 ) ) ;
#13373=PRODUCT_DEFINITION_SHAPE ( 'NONE', 'NONE',  #6723 ) ;
#13527=DIRECTION ( 'NONE',  ( -0.000000000000000000, -1.000000000000000000, -0.000000000000000000 ) ) ;
#13578=DIRECTION ( 'NONE',  ( 0.000000000000000000, 1.000000000000000000, 0.000000000000000000 ) ) ;
#13579=CARTESIAN_POINT ( 'NONE',  ( -15.99999999999979217, -9.000000000000001776, 1.499999999999998890 ) ) ;
#13629=ORIENTED_EDGE ( 'NONE', *, *, #3102, .F. ) ;
#13740=DIRECTION ( 'NONE',  ( 0.000000000000000000, 1.000000000000000000, 0.000000000000000000 ) ) ;
#13742=ORIENTED_EDGE ( 'NONE', *, *, #119, .T. ) ;
#13767=FACE_OUTER_BOUND ( 'NONE', #10859, .T. ) ;
#13832=CLOSED_SHELL ( 'NONE', ( #12367, #10546, #3810, #15812, #13134, #14134, #14069, #12348, #4031, #8354, #763, #3332, #18, #14272 ) ) ;
#13885=EDGE_CURVE ( 'NONE', #6744, #11827, #8399, .T. ) ;
#13890=VECTOR ( 'NONE', #3413, 1000.000000000000000 ) ;
#13896=CARTESIAN_POINT ( 'NONE',  ( -43.99999999999978684, -9.000000000000001776, 1.499999999999998668 ) ) ;
#13914=FACE_OUTER_BOUND ( 'NONE', #11975, .T. ) ;
#13932=CARTESIAN_POINT ( 'NONE',  ( -41.99999999999978684, -9.000000000000001776, 1.499999999999999112 ) ) ;
#13940=EDGE_CURVE ( 'NONE', #13189, #9048, #4783, .T. ) ;
#13997=DIRECTION ( 'NONE',  ( -1.000000000000000000, 0.000000000000000000, 0.000000000000000000 ) ) ;
#14023=DIRECTION ( 'NONE',  ( -0.000000000000000000, -0.000000000000000000, -1.000000000000000000 ) ) ;
#14026=LINE ( 'NONE', #9044, #9624 ) ;
#14036=EDGE_LOOP ( 'NONE', ( #6995, #11702, #454, #4426 ) ) ;
#14069=ADVANCED_FACE ( 'NONE', ( #4065 ), #3256, .T. ) ;
#14071=AXIS2_PLACEMENT_3D ( 'NONE', #13250, #8440, #2039 ) ;
#14077=ORIENTED_EDGE ( 'NONE', *, *, #7809, .F. ) ;
#14134=ADVANCED_FACE ( 'NONE', ( #10308 ), #6668, .F. ) ;
#14145=AXIS2_PLACEMENT_3D ( 'NONE', #5516, #5440, #13009 ) ;
#14183=CARTESIAN_POINT ( 'NONE',  ( -41.99999999999978684, -9.000000000000001776, 3.499999999999998668 ) ) ;
#14199=CARTESIAN_POINT ( 'NONE',  ( -41.99999999999978684, -9.000000000000001776, -3.500000000000000888 ) ) ;
#14230=ORIENTED_EDGE ( 'NONE', *, *, #2350, .F. ) ;
#14264=DIRECTION ( 'NONE',  ( 0.000000000000000000, 0.000000000000000000, -1.000000000000000000 ) ) ;
#14272=ADVANCED_FACE ( 'NONE', ( #15787 ), #914, .F. ) ;
#14291=EDGE_CURVE ( 'NONE', #12397, #5431, #7889, .T. ) ;
#14341=CARTESIAN_POINT ( 'NONE',  ( -43.99999999999978684, -9.000000000000001776, -1.500000000000000666 ) ) ;
#14347=CYLINDRICAL_SURFACE ( 'NONE', #5843, 2.500000000000909495 ) ;
#14406=( LENGTH_UNIT ( ) NAMED_UNIT ( * ) SI_UNIT ( .MILLI., .METRE. ) );
#14483=EDGE_LOOP ( 'NONE', ( #9675, #1193, #1974, #4410 ) ) ;
#14507=LINE ( 'NONE', #7009, #1518 ) ;
#14528=EDGE_CURVE ( 'NONE', #9656, #6965, #9933, .T. ) ;
#14546=CARTESIAN_POINT ( 'NONE',  ( -19.99999999999956657, -9.000000000000001776, 8.786575603324269439E-13 ) ) ;
#14572=AXIS2_PLACEMENT_3D ( 'NONE', #1010, #15806, #6186 ) ;
#14577=DIRECTION ( 'NONE',  ( 0.000000000000000000, 1.000000000000000000, 0.000000000000000000 ) ) ;
#14586=( LENGTH_UNIT ( ) NAMED_UNIT ( * ) SI_UNIT ( .MILLI., .METRE. ) );
#14600=AXIS2_PLACEMENT_3D ( 'NONE', #2728, #6624, #8810 ) ;
#14630=DIRECTION ( 'NONE',  ( 0.000000000000000000, 0.000000000000000000, 1.000000000000000000 ) ) ;
#14673=( NAMED_UNIT ( * ) PLANE_ANGLE_UNIT ( ) SI_UNIT ( $, .RADIAN. ) );
#14724=VERTEX_POINT ( 'NONE', #12192 ) ;
#14748=CARTESIAN_POINT ( 'NONE',  ( -41.99999999999978684, -9.000000000000001776, 3.499999999999998668 ) ) ;
#14813=EDGE_LOOP ( 'NONE', ( #7308, #7785 ) ) ;
#14849=DIRECTION ( 'NONE',  ( -0.000000000000000000, -0.000000000000000000, -1.000000000000000000 ) ) ;
#14934=VECTOR ( 'NONE', #4878, 1000.000000000000000 ) ;
#14936=LINE ( 'NONE', #2875, #6529 ) ;
#14986=DIRECTION ( 'NONE',  ( 0.000000000000000000, 1.000000000000000000, 0.000000000000000000 ) ) ;
#15021=CARTESIAN_POINT ( 'NONE',  ( -17.99999999999979394, -11.00000000000000178, -1.500000000000000888 ) ) ;
#15112=CYLINDRICAL_SURFACE ( 'NONE', #5227, 2.000000000000000888 ) ;
#15130=SHAPE_REPRESENTATION ( 'connector', ( #3223 ), #1938 ) ;
#15198=AXIS2_PLACEMENT_3D ( 'NONE', #2336, #15928, #2254 ) ;
#15217=EDGE_CURVE ( 'NONE', #14724, #307, #8931, .T. ) ;
#15247=PLANE ( 'NONE',  #4263 ) ;
#15310=AXIS2_PLACEMENT_3D ( 'NONE', #9732, #3428, #9574 ) ;
#15349=CARTESIAN_POINT ( 'NONE',  ( -19.99999999999956657, -11.00000000000000178, 2.500000000000877520 ) ) ;
#15355=CARTESIAN_POINT ( 'NONE',  ( -43.99999999999978684, -9.000000000000001776, -1.500000000000000666 ) ) ;
#15383=( LENGTH_UNIT ( ) NAMED_UNIT ( * ) SI_UNIT ( .MILLI., .METRE. ) );
#15487=DIRECTION ( 'NONE',  ( 0.000000000000000000, 0.000000000000000000, 1.000000000000000000 ) ) ;
#15527=ORIENTED_EDGE ( 'NONE', *, *, #15905, .T. ) ;
#15549=ORIENTED_EDGE ( 'NONE', *, *, #1759, .T. ) ;
#15552=DIRECTION ( 'NONE',  ( -0.000000000000000000, -1.000000000000000000, -0.000000000000000000 ) ) ;
#15607=CIRCLE ( 'NONE', #11963, 2.000000000000000888 ) ;
#15727=LINE ( 'NONE', #14341, #12759 ) ;
#15787=FACE_OUTER_BOUND ( 'NONE', #14483, .T. ) ;
#15806=DIRECTION ( 'NONE',  ( 0.000000000000000000, 1.000000000000000000, 0.000000000000000000 ) ) ;
#15812=ADVANCED_FACE ( 'NONE', ( #13767, #2701, #4156 ), #15247, .F. ) ;
#15891=APPLICATION_CONTEXT ( 'automotive_design' ) ;
#15902=DIRECTION ( 'NONE',  ( -0.000000000000000000, -1.000000000000000000, -0.000000000000000000 ) ) ;
#15905=EDGE_CURVE ( 'NONE', #1506, #4542, #15727, .T. ) ;
#15928=DIRECTION ( 'NONE',  ( 0.000000000000000000, 1.000000000000000000, 0.000000000000000000 ) ) ;
ENDSEC;
END-ISO-10303-21;
